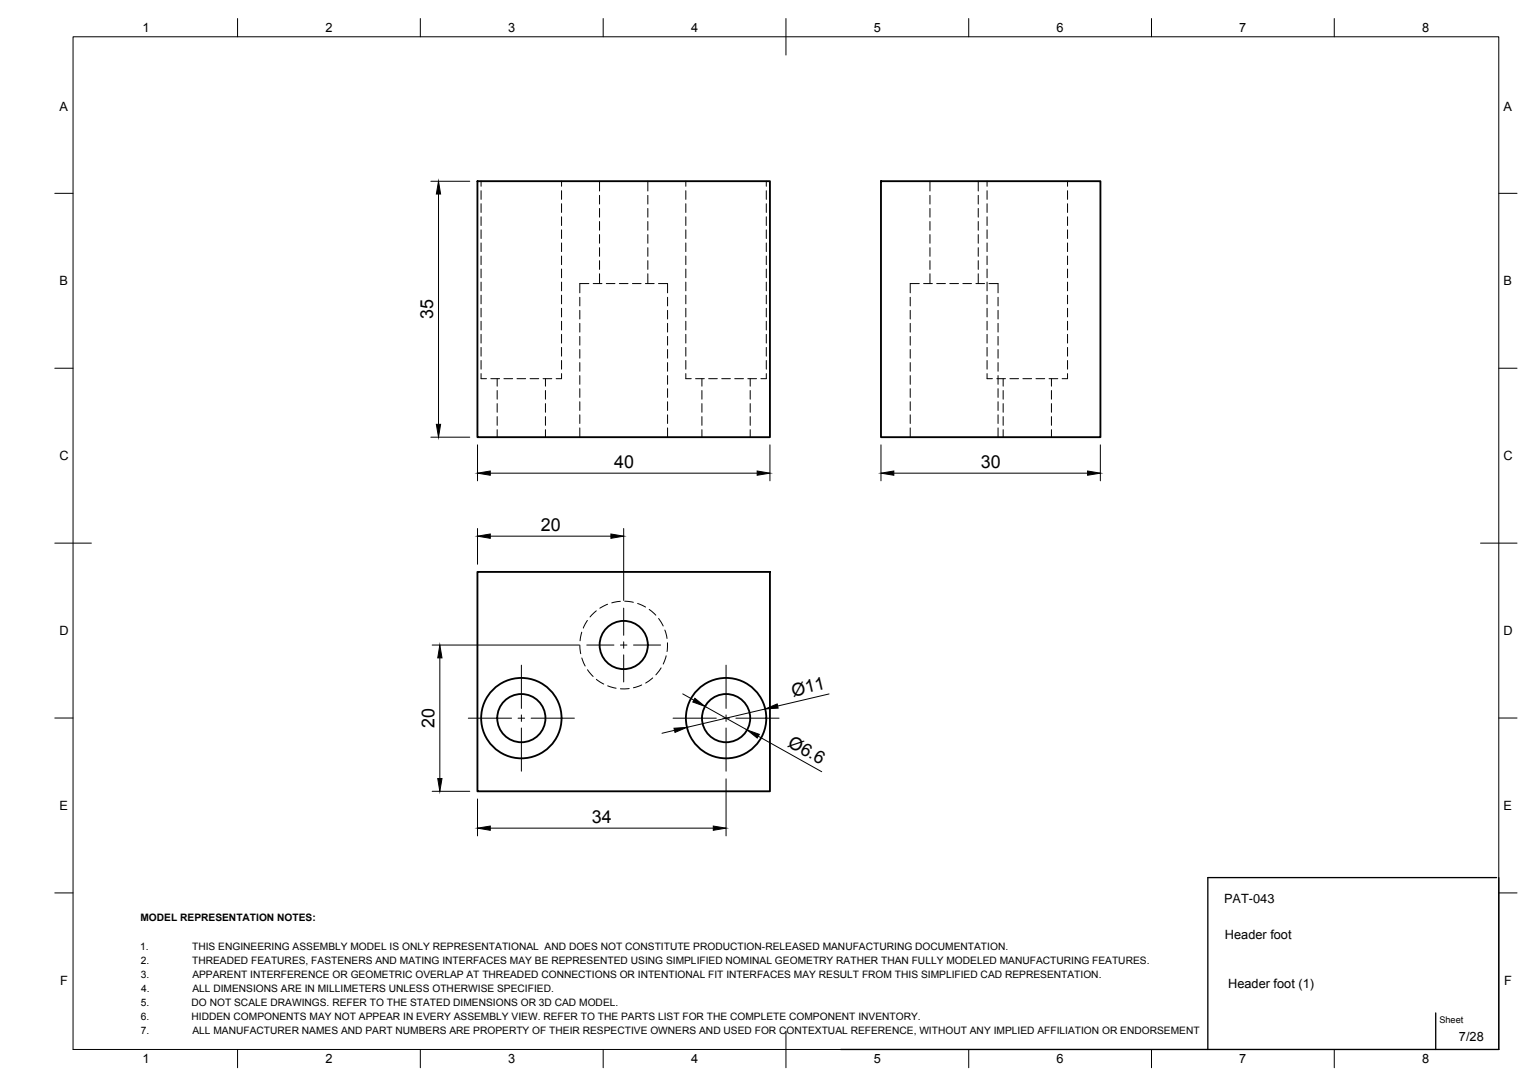
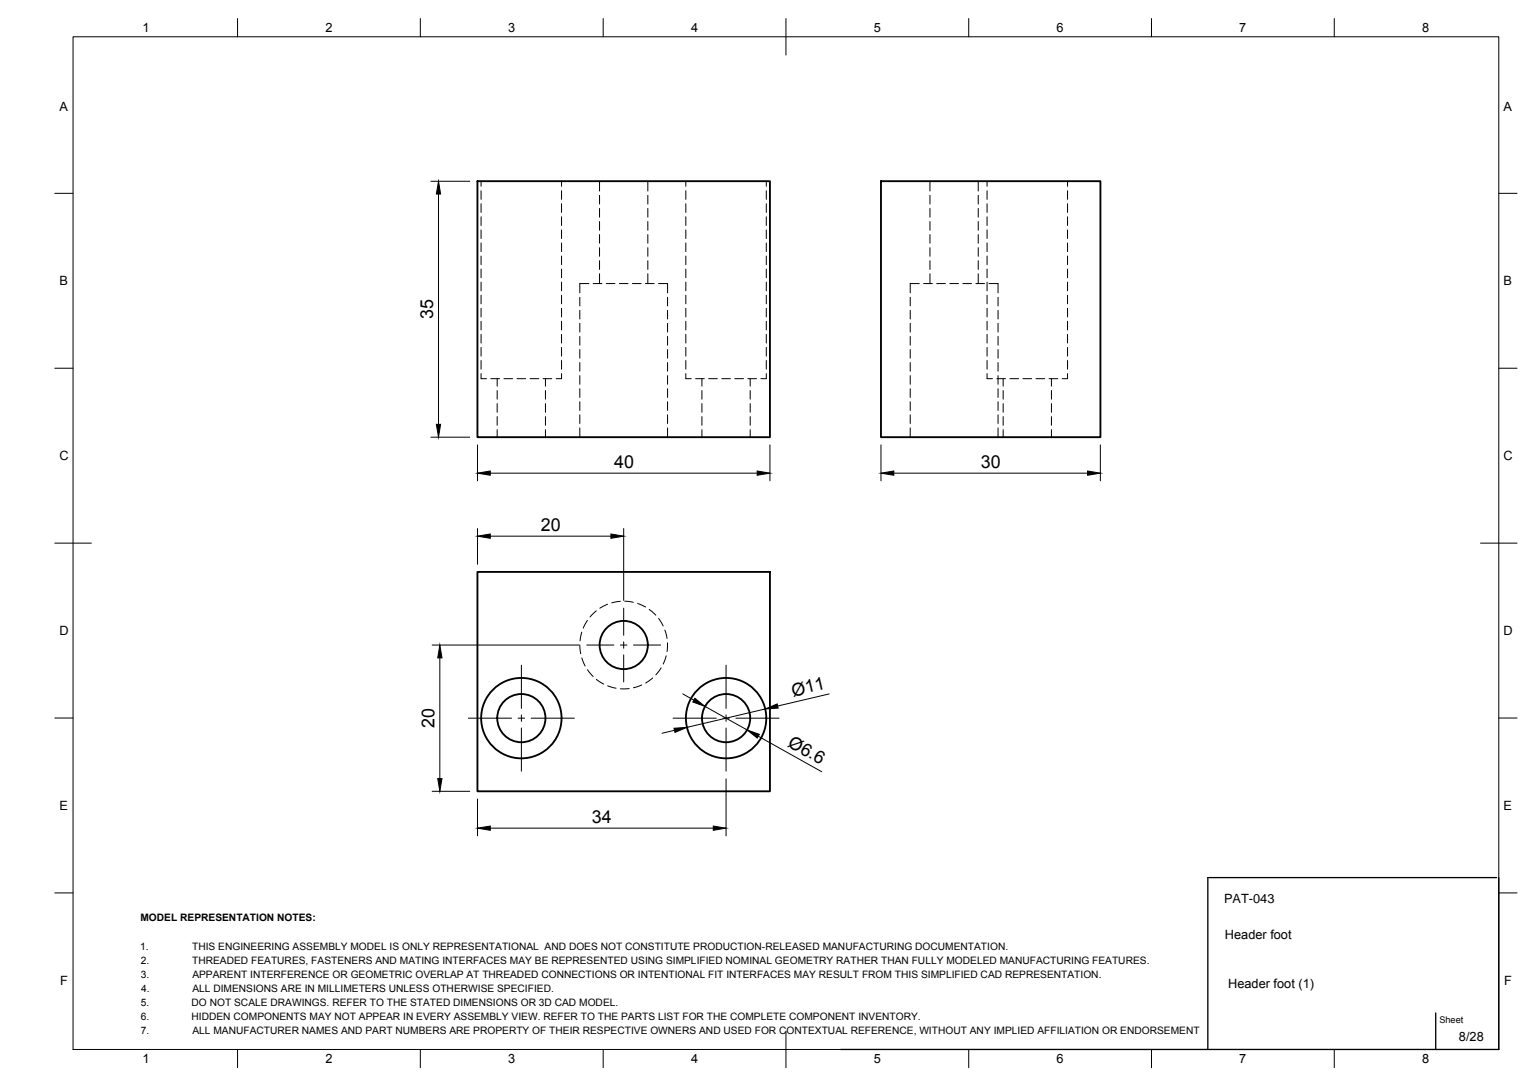
ISO-10303-21;
HEADER;
/* Generated by software containing ST-Developer
 * from STEP Tools, Inc. (www.steptools.com) 
 */

FILE_DESCRIPTION(
/* description */ ('Four-valve pipe header'),
/* implementation_level */ '2;1');

FILE_NAME(
/* name */ 'Header foot (1).step',
/* time_stamp */ '2026-10-29T16:56:19-07:00',
/* author */ (''),
/* organization */ (''),
/* preprocessor_version */ 'ST-DEVELOPER v20.2',
/* originating_system */ 'Autodesk Translation Framework v15.17.0.0',
/* authorisation */ '');

FILE_SCHEMA (('AUTOMOTIVE_DESIGN { 1 0 10303 214 3 1 1 }'));
ENDSEC;

DATA;
#10=MECHANICAL_DESIGN_GEOMETRIC_PRESENTATION_REPRESENTATION('',(#336),#10119);
#284=SHAPE_REPRESENTATION_RELATIONSHIP('SRR','None',#10245,#310);
#310=ADVANCED_BREP_SHAPE_REPRESENTATION('',(#362),#10094);
#336=STYLED_ITEM('',(#10463),#362);
#362=MANIFOLD_SOLID_BREP('Body1',#5582);
#446=FACE_BOUND('',#1177,.T.);
#447=FACE_BOUND('',#1181,.T.);
#448=FACE_BOUND('',#1185,.T.);
#449=FACE_BOUND('',#1192,.T.);
#450=FACE_BOUND('',#1193,.T.);
#451=FACE_BOUND('',#1194,.T.);
#452=FACE_BOUND('',#1196,.T.);
#453=FACE_BOUND('',#1197,.T.);
#454=FACE_BOUND('',#1198,.T.);
#579=PLANE('',#6064);
#580=PLANE('',#6071);
#581=PLANE('',#6078);
#582=PLANE('',#6082);
#583=PLANE('',#6083);
#584=PLANE('',#6084);
#585=PLANE('',#6085);
#586=PLANE('',#6086);
#587=PLANE('',#6087);
#823=FACE_OUTER_BOUND('',#1175,.T.);
#824=FACE_OUTER_BOUND('',#1176,.T.);
#825=FACE_OUTER_BOUND('',#1178,.T.);
#826=FACE_OUTER_BOUND('',#1179,.T.);
#827=FACE_OUTER_BOUND('',#1180,.T.);
#828=FACE_OUTER_BOUND('',#1182,.T.);
#829=FACE_OUTER_BOUND('',#1183,.T.);
#830=FACE_OUTER_BOUND('',#1184,.T.);
#831=FACE_OUTER_BOUND('',#1186,.T.);
#832=FACE_OUTER_BOUND('',#1187,.T.);
#833=FACE_OUTER_BOUND('',#1188,.T.);
#834=FACE_OUTER_BOUND('',#1189,.T.);
#835=FACE_OUTER_BOUND('',#1190,.T.);
#836=FACE_OUTER_BOUND('',#1191,.T.);
#837=FACE_OUTER_BOUND('',#1195,.T.);
#1175=EDGE_LOOP('',(#4105,#4106,#4107,#4108));
#1176=EDGE_LOOP('',(#4109));
#1177=EDGE_LOOP('',(#4110));
#1178=EDGE_LOOP('',(#4111,#4112,#4113,#4114));
#1179=EDGE_LOOP('',(#4115,#4116,#4117,#4118));
#1180=EDGE_LOOP('',(#4119));
#1181=EDGE_LOOP('',(#4120));
#1182=EDGE_LOOP('',(#4121,#4122,#4123,#4124));
#1183=EDGE_LOOP('',(#4125,#4126,#4127,#4128));
#1184=EDGE_LOOP('',(#4129));
#1185=EDGE_LOOP('',(#4130));
#1186=EDGE_LOOP('',(#4131,#4132,#4133,#4134));
#1187=EDGE_LOOP('',(#4135,#4136,#4137,#4138));
#1188=EDGE_LOOP('',(#4139,#4140,#4141,#4142));
#1189=EDGE_LOOP('',(#4143,#4144,#4145,#4146));
#1190=EDGE_LOOP('',(#4147,#4148,#4149,#4150));
#1191=EDGE_LOOP('',(#4151,#4152,#4153,#4154));
#1192=EDGE_LOOP('',(#4155));
#1193=EDGE_LOOP('',(#4156));
#1194=EDGE_LOOP('',(#4157));
#1195=EDGE_LOOP('',(#4158,#4159,#4160,#4161));
#1196=EDGE_LOOP('',(#4162));
#1197=EDGE_LOOP('',(#4163));
#1198=EDGE_LOOP('',(#4164));
#1606=LINE('',#8827,#2024);
#1607=LINE('',#8835,#2025);
#1608=LINE('',#8840,#2026);
#1609=LINE('',#8848,#2027);
#1610=LINE('',#8853,#2028);
#1611=LINE('',#8860,#2029);
#1612=LINE('',#8865,#2030);
#1613=LINE('',#8867,#2031);
#1614=LINE('',#8869,#2032);
#1615=LINE('',#8870,#2033);
#1616=LINE('',#8873,#2034);
#1617=LINE('',#8875,#2035);
#1618=LINE('',#8876,#2036);
#1619=LINE('',#8879,#2037);
#1620=LINE('',#8881,#2038);
#1621=LINE('',#8882,#2039);
#1622=LINE('',#8884,#2040);
#1623=LINE('',#8885,#2041);
#2024=VECTOR('',#6991,0.549999999999997);
#2025=VECTOR('',#7002,0.329999999999998);
#2026=VECTOR('',#7007,0.549999999999997);
#2027=VECTOR('',#7018,0.329999999999998);
#2028=VECTOR('',#7023,0.600000000000001);
#2029=VECTOR('',#7032,0.329999999999998);
#2030=VECTOR('',#7037,1.);
#2031=VECTOR('',#7038,1.);
#2032=VECTOR('',#7039,1.);
#2033=VECTOR('',#7040,1.);
#2034=VECTOR('',#7043,1.);
#2035=VECTOR('',#7044,1.);
#2036=VECTOR('',#7045,1.);
#2037=VECTOR('',#7048,1.);
#2038=VECTOR('',#7049,1.);
#2039=VECTOR('',#7050,1.);
#2040=VECTOR('',#7053,1.);
#2041=VECTOR('',#7054,1.);
#2408=CIRCLE('',#6062,0.549999999999997);
#2409=CIRCLE('',#6063,0.549999999999997);
#2410=CIRCLE('',#6065,0.329999999999998);
#2411=CIRCLE('',#6067,0.329999999999998);
#2412=CIRCLE('',#6069,0.549999999999997);
#2413=CIRCLE('',#6070,0.549999999999997);
#2414=CIRCLE('',#6072,0.329999999999998);
#2415=CIRCLE('',#6074,0.329999999999998);
#2416=CIRCLE('',#6076,0.600000000000001);
#2417=CIRCLE('',#6077,0.600000000000001);
#2418=CIRCLE('',#6079,0.329999999999998);
#2419=CIRCLE('',#6081,0.329999999999998);
#2696=VERTEX_POINT('',#8824);
#2697=VERTEX_POINT('',#8826);
#2698=VERTEX_POINT('',#8830);
#2699=VERTEX_POINT('',#8833);
#2700=VERTEX_POINT('',#8837);
#2701=VERTEX_POINT('',#8839);
#2702=VERTEX_POINT('',#8843);
#2703=VERTEX_POINT('',#8846);
#2704=VERTEX_POINT('',#8850);
#2705=VERTEX_POINT('',#8852);
#2706=VERTEX_POINT('',#8856);
#2707=VERTEX_POINT('',#8859);
#2708=VERTEX_POINT('',#8863);
#2709=VERTEX_POINT('',#8864);
#2710=VERTEX_POINT('',#8866);
#2711=VERTEX_POINT('',#8868);
#2712=VERTEX_POINT('',#8872);
#2713=VERTEX_POINT('',#8874);
#2714=VERTEX_POINT('',#8878);
#2715=VERTEX_POINT('',#8880);
#3219=EDGE_CURVE('',#2696,#2696,#2408,.T.);
#3220=EDGE_CURVE('',#2696,#2697,#1606,.T.);
#3221=EDGE_CURVE('',#2697,#2697,#2409,.T.);
#3222=EDGE_CURVE('',#2698,#2698,#2410,.T.);
#3223=EDGE_CURVE('',#2699,#2699,#2411,.T.);
#3224=EDGE_CURVE('',#2699,#2698,#1607,.T.);
#3225=EDGE_CURVE('',#2700,#2700,#2412,.T.);
#3226=EDGE_CURVE('',#2700,#2701,#1608,.T.);
#3227=EDGE_CURVE('',#2701,#2701,#2413,.T.);
#3228=EDGE_CURVE('',#2702,#2702,#2414,.T.);
#3229=EDGE_CURVE('',#2703,#2703,#2415,.T.);
#3230=EDGE_CURVE('',#2703,#2702,#1609,.T.);
#3231=EDGE_CURVE('',#2704,#2704,#2416,.T.);
#3232=EDGE_CURVE('',#2704,#2705,#1610,.T.);
#3233=EDGE_CURVE('',#2705,#2705,#2417,.T.);
#3234=EDGE_CURVE('',#2706,#2706,#2418,.T.);
#3235=EDGE_CURVE('',#2706,#2707,#1611,.T.);
#3236=EDGE_CURVE('',#2707,#2707,#2419,.T.);
#3237=EDGE_CURVE('',#2708,#2709,#1612,.T.);
#3238=EDGE_CURVE('',#2709,#2710,#1613,.T.);
#3239=EDGE_CURVE('',#2711,#2710,#1614,.T.);
#3240=EDGE_CURVE('',#2708,#2711,#1615,.T.);
#3241=EDGE_CURVE('',#2712,#2708,#1616,.T.);
#3242=EDGE_CURVE('',#2713,#2711,#1617,.T.);
#3243=EDGE_CURVE('',#2712,#2713,#1618,.T.);
#3244=EDGE_CURVE('',#2714,#2712,#1619,.T.);
#3245=EDGE_CURVE('',#2715,#2713,#1620,.T.);
#3246=EDGE_CURVE('',#2714,#2715,#1621,.T.);
#3247=EDGE_CURVE('',#2709,#2714,#1622,.T.);
#3248=EDGE_CURVE('',#2710,#2715,#1623,.T.);
#4105=ORIENTED_EDGE('',*,*,#3219,.F.);
#4106=ORIENTED_EDGE('',*,*,#3220,.T.);
#4107=ORIENTED_EDGE('',*,*,#3221,.F.);
#4108=ORIENTED_EDGE('',*,*,#3220,.F.);
#4109=ORIENTED_EDGE('',*,*,#3219,.T.);
#4110=ORIENTED_EDGE('',*,*,#3222,.F.);
#4111=ORIENTED_EDGE('',*,*,#3223,.F.);
#4112=ORIENTED_EDGE('',*,*,#3224,.T.);
#4113=ORIENTED_EDGE('',*,*,#3222,.T.);
#4114=ORIENTED_EDGE('',*,*,#3224,.F.);
#4115=ORIENTED_EDGE('',*,*,#3225,.F.);
#4116=ORIENTED_EDGE('',*,*,#3226,.T.);
#4117=ORIENTED_EDGE('',*,*,#3227,.F.);
#4118=ORIENTED_EDGE('',*,*,#3226,.F.);
#4119=ORIENTED_EDGE('',*,*,#3225,.T.);
#4120=ORIENTED_EDGE('',*,*,#3228,.F.);
#4121=ORIENTED_EDGE('',*,*,#3229,.F.);
#4122=ORIENTED_EDGE('',*,*,#3230,.T.);
#4123=ORIENTED_EDGE('',*,*,#3228,.T.);
#4124=ORIENTED_EDGE('',*,*,#3230,.F.);
#4125=ORIENTED_EDGE('',*,*,#3231,.F.);
#4126=ORIENTED_EDGE('',*,*,#3232,.T.);
#4127=ORIENTED_EDGE('',*,*,#3233,.T.);
#4128=ORIENTED_EDGE('',*,*,#3232,.F.);
#4129=ORIENTED_EDGE('',*,*,#3233,.F.);
#4130=ORIENTED_EDGE('',*,*,#3234,.F.);
#4131=ORIENTED_EDGE('',*,*,#3234,.T.);
#4132=ORIENTED_EDGE('',*,*,#3235,.T.);
#4133=ORIENTED_EDGE('',*,*,#3236,.F.);
#4134=ORIENTED_EDGE('',*,*,#3235,.F.);
#4135=ORIENTED_EDGE('',*,*,#3237,.T.);
#4136=ORIENTED_EDGE('',*,*,#3238,.T.);
#4137=ORIENTED_EDGE('',*,*,#3239,.F.);
#4138=ORIENTED_EDGE('',*,*,#3240,.F.);
#4139=ORIENTED_EDGE('',*,*,#3241,.T.);
#4140=ORIENTED_EDGE('',*,*,#3240,.T.);
#4141=ORIENTED_EDGE('',*,*,#3242,.F.);
#4142=ORIENTED_EDGE('',*,*,#3243,.F.);
#4143=ORIENTED_EDGE('',*,*,#3244,.T.);
#4144=ORIENTED_EDGE('',*,*,#3243,.T.);
#4145=ORIENTED_EDGE('',*,*,#3245,.F.);
#4146=ORIENTED_EDGE('',*,*,#3246,.F.);
#4147=ORIENTED_EDGE('',*,*,#3247,.T.);
#4148=ORIENTED_EDGE('',*,*,#3246,.T.);
#4149=ORIENTED_EDGE('',*,*,#3248,.F.);
#4150=ORIENTED_EDGE('',*,*,#3238,.F.);
#4151=ORIENTED_EDGE('',*,*,#3248,.T.);
#4152=ORIENTED_EDGE('',*,*,#3245,.T.);
#4153=ORIENTED_EDGE('',*,*,#3242,.T.);
#4154=ORIENTED_EDGE('',*,*,#3239,.T.);
#4155=ORIENTED_EDGE('',*,*,#3221,.T.);
#4156=ORIENTED_EDGE('',*,*,#3227,.T.);
#4157=ORIENTED_EDGE('',*,*,#3236,.T.);
#4158=ORIENTED_EDGE('',*,*,#3247,.F.);
#4159=ORIENTED_EDGE('',*,*,#3237,.F.);
#4160=ORIENTED_EDGE('',*,*,#3241,.F.);
#4161=ORIENTED_EDGE('',*,*,#3244,.F.);
#4162=ORIENTED_EDGE('',*,*,#3223,.T.);
#4163=ORIENTED_EDGE('',*,*,#3229,.T.);
#4164=ORIENTED_EDGE('',*,*,#3231,.T.);
#5181=CYLINDRICAL_SURFACE('',#6061,0.549999999999997);
#5182=CYLINDRICAL_SURFACE('',#6066,0.329999999999998);
#5183=CYLINDRICAL_SURFACE('',#6068,0.549999999999997);
#5184=CYLINDRICAL_SURFACE('',#6073,0.329999999999998);
#5185=CYLINDRICAL_SURFACE('',#6075,0.600000000000001);
#5186=CYLINDRICAL_SURFACE('',#6080,0.329999999999998);
#5323=ADVANCED_FACE('',(#823),#5181,.F.);
#5324=ADVANCED_FACE('',(#824,#446),#579,.T.);
#5325=ADVANCED_FACE('',(#825),#5182,.F.);
#5326=ADVANCED_FACE('',(#826),#5183,.F.);
#5327=ADVANCED_FACE('',(#827,#447),#580,.T.);
#5328=ADVANCED_FACE('',(#828),#5184,.F.);
#5329=ADVANCED_FACE('',(#829),#5185,.F.);
#5330=ADVANCED_FACE('',(#830,#448),#581,.F.);
#5331=ADVANCED_FACE('',(#831),#5186,.F.);
#5332=ADVANCED_FACE('',(#832),#582,.T.);
#5333=ADVANCED_FACE('',(#833),#583,.T.);
#5334=ADVANCED_FACE('',(#834),#584,.T.);
#5335=ADVANCED_FACE('',(#835),#585,.T.);
#5336=ADVANCED_FACE('',(#836,#449,#450,#451),#586,.T.);
#5337=ADVANCED_FACE('',(#837,#452,#453,#454),#587,.F.);
#5582=CLOSED_SHELL('',(#5323,#5324,#5325,#5326,#5327,#5328,#5329,#5330,
#5331,#5332,#5333,#5334,#5335,#5336,#5337));
#6060=AXIS2_PLACEMENT_3D('',#8822,#6985,#6986);
#6061=AXIS2_PLACEMENT_3D('',#8823,#6987,#6988);
#6062=AXIS2_PLACEMENT_3D('',#8825,#6989,#6990);
#6063=AXIS2_PLACEMENT_3D('',#8828,#6992,#6993);
#6064=AXIS2_PLACEMENT_3D('',#8829,#6994,#6995);
#6065=AXIS2_PLACEMENT_3D('',#8831,#6996,#6997);
#6066=AXIS2_PLACEMENT_3D('',#8832,#6998,#6999);
#6067=AXIS2_PLACEMENT_3D('',#8834,#7000,#7001);
#6068=AXIS2_PLACEMENT_3D('',#8836,#7003,#7004);
#6069=AXIS2_PLACEMENT_3D('',#8838,#7005,#7006);
#6070=AXIS2_PLACEMENT_3D('',#8841,#7008,#7009);
#6071=AXIS2_PLACEMENT_3D('',#8842,#7010,#7011);
#6072=AXIS2_PLACEMENT_3D('',#8844,#7012,#7013);
#6073=AXIS2_PLACEMENT_3D('',#8845,#7014,#7015);
#6074=AXIS2_PLACEMENT_3D('',#8847,#7016,#7017);
#6075=AXIS2_PLACEMENT_3D('',#8849,#7019,#7020);
#6076=AXIS2_PLACEMENT_3D('',#8851,#7021,#7022);
#6077=AXIS2_PLACEMENT_3D('',#8854,#7024,#7025);
#6078=AXIS2_PLACEMENT_3D('',#8855,#7026,#7027);
#6079=AXIS2_PLACEMENT_3D('',#8857,#7028,#7029);
#6080=AXIS2_PLACEMENT_3D('',#8858,#7030,#7031);
#6081=AXIS2_PLACEMENT_3D('',#8861,#7033,#7034);
#6082=AXIS2_PLACEMENT_3D('',#8862,#7035,#7036);
#6083=AXIS2_PLACEMENT_3D('',#8871,#7041,#7042);
#6084=AXIS2_PLACEMENT_3D('',#8877,#7046,#7047);
#6085=AXIS2_PLACEMENT_3D('',#8883,#7051,#7052);
#6086=AXIS2_PLACEMENT_3D('',#8886,#7055,#7056);
#6087=AXIS2_PLACEMENT_3D('',#8887,#7057,#7058);
#6985=DIRECTION('axis',(0.,0.,1.));
#6986=DIRECTION('refdir',(1.,0.,0.));
#6987=DIRECTION('center_axis',(0.,0.,1.));
#6988=DIRECTION('ref_axis',(1.,0.,0.));
#6989=DIRECTION('center_axis',(0.,0.,1.));
#6990=DIRECTION('ref_axis',(1.,0.,0.));
#6991=DIRECTION('',(0.,0.,1.));
#6992=DIRECTION('center_axis',(0.,0.,-1.));
#6993=DIRECTION('ref_axis',(1.,0.,0.));
#6994=DIRECTION('center_axis',(0.,0.,1.));
#6995=DIRECTION('ref_axis',(1.,0.,0.));
#6996=DIRECTION('center_axis',(0.,0.,1.));
#6997=DIRECTION('ref_axis',(1.,0.,0.));
#6998=DIRECTION('center_axis',(0.,0.,1.));
#6999=DIRECTION('ref_axis',(1.,0.,0.));
#7000=DIRECTION('center_axis',(0.,0.,1.));
#7001=DIRECTION('ref_axis',(1.,0.,0.));
#7002=DIRECTION('',(0.,0.,1.));
#7003=DIRECTION('center_axis',(0.,0.,1.));
#7004=DIRECTION('ref_axis',(1.,0.,0.));
#7005=DIRECTION('center_axis',(0.,0.,1.));
#7006=DIRECTION('ref_axis',(1.,0.,0.));
#7007=DIRECTION('',(0.,0.,1.));
#7008=DIRECTION('center_axis',(0.,0.,-1.));
#7009=DIRECTION('ref_axis',(1.,0.,0.));
#7010=DIRECTION('center_axis',(0.,0.,1.));
#7011=DIRECTION('ref_axis',(1.,0.,0.));
#7012=DIRECTION('center_axis',(0.,0.,1.));
#7013=DIRECTION('ref_axis',(1.,0.,0.));
#7014=DIRECTION('center_axis',(0.,0.,1.));
#7015=DIRECTION('ref_axis',(1.,0.,0.));
#7016=DIRECTION('center_axis',(0.,0.,1.));
#7017=DIRECTION('ref_axis',(1.,0.,0.));
#7018=DIRECTION('',(0.,0.,1.));
#7019=DIRECTION('center_axis',(0.,0.,1.));
#7020=DIRECTION('ref_axis',(1.,0.,0.));
#7021=DIRECTION('center_axis',(0.,0.,1.));
#7022=DIRECTION('ref_axis',(1.,0.,0.));
#7023=DIRECTION('',(0.,0.,1.));
#7024=DIRECTION('center_axis',(0.,0.,1.));
#7025=DIRECTION('ref_axis',(1.,0.,0.));
#7026=DIRECTION('center_axis',(0.,0.,1.));
#7027=DIRECTION('ref_axis',(1.,0.,0.));
#7028=DIRECTION('center_axis',(0.,0.,-1.));
#7029=DIRECTION('ref_axis',(1.,0.,0.));
#7030=DIRECTION('center_axis',(0.,0.,1.));
#7031=DIRECTION('ref_axis',(1.,0.,0.));
#7032=DIRECTION('',(0.,0.,1.));
#7033=DIRECTION('center_axis',(0.,0.,-1.));
#7034=DIRECTION('ref_axis',(1.,0.,0.));
#7035=DIRECTION('center_axis',(0.,1.,0.));
#7036=DIRECTION('ref_axis',(-1.,0.,0.));
#7037=DIRECTION('',(-1.,0.,0.));
#7038=DIRECTION('',(0.,0.,1.));
#7039=DIRECTION('',(-1.,0.,0.));
#7040=DIRECTION('',(0.,0.,1.));
#7041=DIRECTION('center_axis',(1.,0.,0.));
#7042=DIRECTION('ref_axis',(0.,1.,0.));
#7043=DIRECTION('',(0.,1.,0.));
#7044=DIRECTION('',(0.,1.,0.));
#7045=DIRECTION('',(0.,0.,1.));
#7046=DIRECTION('center_axis',(0.,-1.,0.));
#7047=DIRECTION('ref_axis',(1.,0.,0.));
#7048=DIRECTION('',(1.,0.,0.));
#7049=DIRECTION('',(1.,0.,0.));
#7050=DIRECTION('',(0.,0.,1.));
#7051=DIRECTION('center_axis',(-1.,0.,0.));
#7052=DIRECTION('ref_axis',(0.,-1.,0.));
#7053=DIRECTION('',(0.,-1.,0.));
#7054=DIRECTION('',(0.,-1.,0.));
#7055=DIRECTION('center_axis',(0.,0.,1.));
#7056=DIRECTION('ref_axis',(1.,0.,0.));
#7057=DIRECTION('center_axis',(0.,0.,1.));
#7058=DIRECTION('ref_axis',(1.,0.,0.));
#8822=CARTESIAN_POINT('',(0.,0.,0.));
#8823=CARTESIAN_POINT('Origin',(39.9,10.,0.8));
#8824=CARTESIAN_POINT('',(39.35,10.,0.8));
#8825=CARTESIAN_POINT('Origin',(39.9,10.,0.8));
#8826=CARTESIAN_POINT('',(39.35,10.,3.5));
#8827=CARTESIAN_POINT('',(39.35,10.,0.8));
#8828=CARTESIAN_POINT('Origin',(39.9,10.,3.5));
#8829=CARTESIAN_POINT('Origin',(39.9,10.,0.8));
#8830=CARTESIAN_POINT('',(39.57,10.,0.8));
#8831=CARTESIAN_POINT('Origin',(39.9,10.,0.8));
#8832=CARTESIAN_POINT('Origin',(39.9,10.,-0.1));
#8833=CARTESIAN_POINT('',(39.57,10.,0.));
#8834=CARTESIAN_POINT('Origin',(39.9,10.,0.));
#8835=CARTESIAN_POINT('',(39.57,10.,-0.1));
#8836=CARTESIAN_POINT('Origin',(37.1,10.,0.8));
#8837=CARTESIAN_POINT('',(36.55,10.,0.8));
#8838=CARTESIAN_POINT('Origin',(37.1,10.,0.8));
#8839=CARTESIAN_POINT('',(36.55,10.,3.5));
#8840=CARTESIAN_POINT('',(36.55,10.,0.8));
#8841=CARTESIAN_POINT('Origin',(37.1,10.,3.5));
#8842=CARTESIAN_POINT('Origin',(37.1,10.,0.8));
#8843=CARTESIAN_POINT('',(36.77,10.,0.8));
#8844=CARTESIAN_POINT('Origin',(37.1,10.,0.8));
#8845=CARTESIAN_POINT('Origin',(37.1,10.,-0.1));
#8846=CARTESIAN_POINT('',(36.77,10.,0.));
#8847=CARTESIAN_POINT('Origin',(37.1,10.,0.));
#8848=CARTESIAN_POINT('',(36.77,10.,-0.1));
#8849=CARTESIAN_POINT('Origin',(38.5,9.,-0.1));
#8850=CARTESIAN_POINT('',(37.9,9.,0.));
#8851=CARTESIAN_POINT('Origin',(38.5,9.,0.));
#8852=CARTESIAN_POINT('',(37.9,9.,2.1));
#8853=CARTESIAN_POINT('',(37.9,9.,-0.1));
#8854=CARTESIAN_POINT('Origin',(38.5,9.,2.1));
#8855=CARTESIAN_POINT('Origin',(38.5,9.,2.1));
#8856=CARTESIAN_POINT('',(38.17,9.,2.1));
#8857=CARTESIAN_POINT('Origin',(38.5,9.,2.1));
#8858=CARTESIAN_POINT('Origin',(38.5,9.,-0.1));
#8859=CARTESIAN_POINT('',(38.17,9.,3.5));
#8860=CARTESIAN_POINT('',(38.17,9.,-0.1));
#8861=CARTESIAN_POINT('Origin',(38.5,9.,3.5));
#8862=CARTESIAN_POINT('Origin',(40.5,11.,0.));
#8863=CARTESIAN_POINT('',(40.5,11.,0.));
#8864=CARTESIAN_POINT('',(36.5,11.,0.));
#8865=CARTESIAN_POINT('',(40.5,11.,0.));
#8866=CARTESIAN_POINT('',(36.5,11.,3.5));
#8867=CARTESIAN_POINT('',(36.5,11.,0.));
#8868=CARTESIAN_POINT('',(40.5,11.,3.5));
#8869=CARTESIAN_POINT('',(40.5,11.,3.5));
#8870=CARTESIAN_POINT('',(40.5,11.,0.));
#8871=CARTESIAN_POINT('Origin',(40.5,8.,0.));
#8872=CARTESIAN_POINT('',(40.5,8.,0.));
#8873=CARTESIAN_POINT('',(40.5,8.,0.));
#8874=CARTESIAN_POINT('',(40.5,8.,3.5));
#8875=CARTESIAN_POINT('',(40.5,8.,3.5));
#8876=CARTESIAN_POINT('',(40.5,8.,0.));
#8877=CARTESIAN_POINT('Origin',(36.5,8.,0.));
#8878=CARTESIAN_POINT('',(36.5,8.,0.));
#8879=CARTESIAN_POINT('',(36.5,8.,0.));
#8880=CARTESIAN_POINT('',(36.5,8.,3.5));
#8881=CARTESIAN_POINT('',(36.5,8.,3.5));
#8882=CARTESIAN_POINT('',(36.5,8.,0.));
#8883=CARTESIAN_POINT('Origin',(36.5,11.,0.));
#8884=CARTESIAN_POINT('',(36.5,11.,0.));
#8885=CARTESIAN_POINT('',(36.5,11.,3.5));
#8886=CARTESIAN_POINT('Origin',(38.5,9.5,3.5));
#8887=CARTESIAN_POINT('Origin',(38.5,9.5,0.));
#10063=UNCERTAINTY_MEASURE_WITH_UNIT(LENGTH_MEASURE(0.001),#10120,
'DISTANCE_ACCURACY_VALUE',
'Maximum model space distance between geometric entities at asserted c
onnectivities');
#10088=UNCERTAINTY_MEASURE_WITH_UNIT(LENGTH_MEASURE(0.001),#10120,
'DISTANCE_ACCURACY_VALUE',
'Maximum model space distance between geometric entities at asserted c
onnectivities');
#10094=(
GEOMETRIC_REPRESENTATION_CONTEXT(3)
GLOBAL_UNCERTAINTY_ASSIGNED_CONTEXT((#10063))
GLOBAL_UNIT_ASSIGNED_CONTEXT((#10120,#10122,#10123))
REPRESENTATION_CONTEXT('','3D')
);
#10119=(
GEOMETRIC_REPRESENTATION_CONTEXT(3)
GLOBAL_UNCERTAINTY_ASSIGNED_CONTEXT((#10088))
GLOBAL_UNIT_ASSIGNED_CONTEXT((#10120,#10122,#10123))
REPRESENTATION_CONTEXT('','3D')
);
#10120=(
LENGTH_UNIT()
NAMED_UNIT(*)
SI_UNIT(.CENTI.,.METRE.)
);
#10122=(
NAMED_UNIT(*)
PLANE_ANGLE_UNIT()
SI_UNIT($,.RADIAN.)
);
#10123=(
NAMED_UNIT(*)
SI_UNIT($,.STERADIAN.)
SOLID_ANGLE_UNIT()
);
#10129=SHAPE_DEFINITION_REPRESENTATION(#10159,#10245);
#10159=PRODUCT_DEFINITION_SHAPE('',$,#10276);
#10245=SHAPE_REPRESENTATION('',(#6060),#10094);
#10270=PRODUCT_DEFINITION_CONTEXT('part definition',#10362,'design');
#10276=PRODUCT_DEFINITION('Header foot (1)','Header foot (1)',#10306,#10270);
#10306=PRODUCT_DEFINITION_FORMATION('',$,#10369);
#10362=APPLICATION_CONTEXT(
'Core Data for Automotive Mechanical Design Process');
#10363=PRODUCT_CONTEXT('part definition',#10362,'mechanical');
#10369=PRODUCT('Header foot (1)','Header foot (1)','Header foot (1)',(#10363));
#10457=COLOUR_RGB('Sky Blue',0.24,0.69,0.87);
#10458=FILL_AREA_STYLE_COLOUR('',#10457);
#10459=FILL_AREA_STYLE('',(#10458));
#10460=SURFACE_STYLE_FILL_AREA(#10459);
#10461=SURFACE_SIDE_STYLE('',(#10460));
#10462=SURFACE_STYLE_USAGE(.BOTH.,#10461);
#10463=PRESENTATION_STYLE_ASSIGNMENT((#10462));
ENDSEC;
END-ISO-10303-21;
